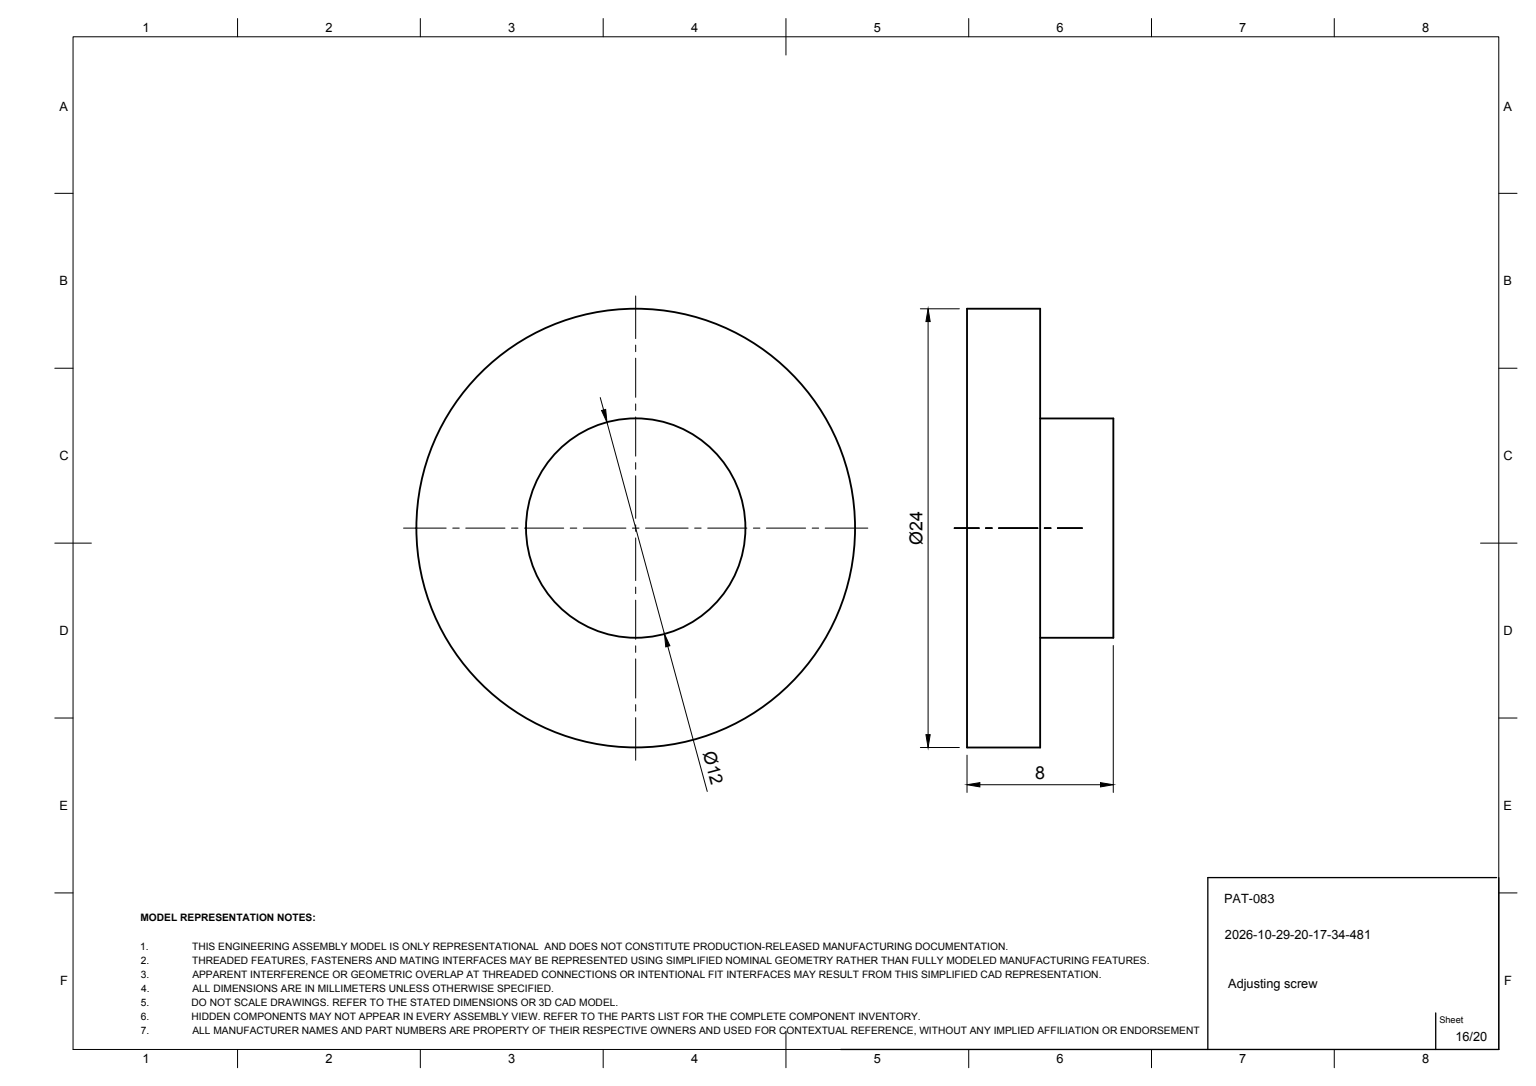
ISO-10303-21;
HEADER;
/* Generated by software containing ST-Developer
 * from STEP Tools, Inc. (www.steptools.com) 
 */

FILE_DESCRIPTION(
/* description */ ('PAT-083'),
/* implementation_level */ '2;1');

FILE_NAME(
/* name */ 'Adjusting screw.step',
/* time_stamp */ '2026-10-29T20:18:00-07:00',
/* author */ (''),
/* organization */ (''),
/* preprocessor_version */ 'ST-DEVELOPER v20.2',
/* originating_system */ 'Autodesk Translation Framework v15.17.0.0',
/* authorisation */ '');

FILE_SCHEMA (('AUTOMOTIVE_DESIGN { 1 0 10303 214 3 1 1 }'));
ENDSEC;

DATA;
#10=MECHANICAL_DESIGN_GEOMETRIC_PRESENTATION_REPRESENTATION('',(#243),#8428);
#195=SHAPE_REPRESENTATION_RELATIONSHIP('SRR','None',#8529,#219);
#219=ADVANCED_BREP_SHAPE_REPRESENTATION('',(#267),#8418);
#243=STYLED_ITEM('',(#8712),#267);
#267=MANIFOLD_SOLID_BREP('Body1',#3689);
#426=PLANE('',#4256);
#427=PLANE('',#4257);
#630=FACE_OUTER_BOUND('',#929,.T.);
#631=FACE_OUTER_BOUND('',#930,.T.);
#632=FACE_OUTER_BOUND('',#931,.T.);
#929=EDGE_LOOP('',(#2978,#2979,#2980,#2981));
#930=EDGE_LOOP('',(#2982));
#931=EDGE_LOOP('',(#2983));
#1153=LINE('',#7851,#1397);
#1397=VECTOR('',#5125,0.4);
#1668=CIRCLE('',#4254,0.4);
#1669=CIRCLE('',#4255,0.4);
#1881=VERTEX_POINT('',#7848);
#1882=VERTEX_POINT('',#7850);
#2265=EDGE_CURVE('',#1881,#1881,#1668,.T.);
#2266=EDGE_CURVE('',#1881,#1882,#1153,.T.);
#2267=EDGE_CURVE('',#1882,#1882,#1669,.T.);
#2978=ORIENTED_EDGE('',*,*,#2265,.F.);
#2979=ORIENTED_EDGE('',*,*,#2266,.T.);
#2980=ORIENTED_EDGE('',*,*,#2267,.T.);
#2981=ORIENTED_EDGE('',*,*,#2266,.F.);
#2982=ORIENTED_EDGE('',*,*,#2265,.T.);
#2983=ORIENTED_EDGE('',*,*,#2267,.F.);
#3427=CYLINDRICAL_SURFACE('',#4253,0.4);
#3577=ADVANCED_FACE('',(#630),#3427,.T.);
#3578=ADVANCED_FACE('',(#631),#426,.T.);
#3579=ADVANCED_FACE('',(#632),#427,.F.);
#3689=CLOSED_SHELL('',(#3577,#3578,#3579));
#4252=AXIS2_PLACEMENT_3D('',#7846,#5119,#5120);
#4253=AXIS2_PLACEMENT_3D('',#7847,#5121,#5122);
#4254=AXIS2_PLACEMENT_3D('',#7849,#5123,#5124);
#4255=AXIS2_PLACEMENT_3D('',#7852,#5126,#5127);
#4256=AXIS2_PLACEMENT_3D('',#7853,#5128,#5129);
#4257=AXIS2_PLACEMENT_3D('',#7854,#5130,#5131);
#5119=DIRECTION('axis',(0.,0.,1.));
#5120=DIRECTION('refdir',(1.,0.,0.));
#5121=DIRECTION('center_axis',(0.,0.,1.));
#5122=DIRECTION('ref_axis',(1.,0.,0.));
#5123=DIRECTION('center_axis',(0.,0.,1.));
#5124=DIRECTION('ref_axis',(1.,0.,0.));
#5125=DIRECTION('',(0.,0.,-1.));
#5126=DIRECTION('center_axis',(0.,0.,1.));
#5127=DIRECTION('ref_axis',(1.,0.,0.));
#5128=DIRECTION('center_axis',(0.,0.,1.));
#5129=DIRECTION('ref_axis',(1.,0.,0.));
#5130=DIRECTION('center_axis',(0.,0.,1.));
#5131=DIRECTION('ref_axis',(1.,0.,0.));
#7846=CARTESIAN_POINT('',(0.,0.,0.));
#7847=CARTESIAN_POINT('Origin',(0.,0.,8.));
#7848=CARTESIAN_POINT('',(-0.4,-4.89858719658941E-17,11.));
#7849=CARTESIAN_POINT('Origin',(0.,0.,11.));
#7850=CARTESIAN_POINT('',(-0.4,-4.89858719658941E-17,8.));
#7851=CARTESIAN_POINT('',(-0.4,-4.89858719658941E-17,8.));
#7852=CARTESIAN_POINT('Origin',(0.,0.,8.));
#7853=CARTESIAN_POINT('Origin',(0.,0.,11.));
#7854=CARTESIAN_POINT('Origin',(0.,0.,8.));
#8392=UNCERTAINTY_MEASURE_WITH_UNIT(LENGTH_MEASURE(0.001),#8429,
'DISTANCE_ACCURACY_VALUE',
'Maximum model space distance between geometric entities at asserted c
onnectivities');
#8402=UNCERTAINTY_MEASURE_WITH_UNIT(LENGTH_MEASURE(0.001),#8429,
'DISTANCE_ACCURACY_VALUE',
'Maximum model space distance between geometric entities at asserted c
onnectivities');
#8418=(
GEOMETRIC_REPRESENTATION_CONTEXT(3)
GLOBAL_UNCERTAINTY_ASSIGNED_CONTEXT((#8392))
GLOBAL_UNIT_ASSIGNED_CONTEXT((#8429,#8431,#8432))
REPRESENTATION_CONTEXT('','3D')
);
#8428=(
GEOMETRIC_REPRESENTATION_CONTEXT(3)
GLOBAL_UNCERTAINTY_ASSIGNED_CONTEXT((#8402))
GLOBAL_UNIT_ASSIGNED_CONTEXT((#8429,#8431,#8432))
REPRESENTATION_CONTEXT('','3D')
);
#8429=(
LENGTH_UNIT()
NAMED_UNIT(*)
SI_UNIT(.CENTI.,.METRE.)
);
#8431=(
NAMED_UNIT(*)
PLANE_ANGLE_UNIT()
SI_UNIT($,.RADIAN.)
);
#8432=(
NAMED_UNIT(*)
SI_UNIT($,.STERADIAN.)
SOLID_ANGLE_UNIT()
);
#8448=SHAPE_DEFINITION_REPRESENTATION(#8473,#8529);
#8473=PRODUCT_DEFINITION_SHAPE('',$,#8555);
#8529=SHAPE_REPRESENTATION('',(#4252),#8418);
#8539=PRODUCT_DEFINITION_CONTEXT('part definition',#8616,'design');
#8555=PRODUCT_DEFINITION('Adjusting screw','Adjusting screw',#8580,
#8539);
#8580=PRODUCT_DEFINITION_FORMATION('',$,#8633);
#8616=APPLICATION_CONTEXT(
'Core Data for Automotive Mechanical Design Process');
#8617=PRODUCT_CONTEXT('part definition',#8616,'mechanical');
#8633=PRODUCT('Adjusting screw','Adjusting screw',
'Adjusting screw',(#8617));
#8706=COLOUR_RGB('Black',0.12,0.14,0.17);
#8707=FILL_AREA_STYLE_COLOUR('',#8706);
#8708=FILL_AREA_STYLE('',(#8707));
#8709=SURFACE_STYLE_FILL_AREA(#8708);
#8710=SURFACE_SIDE_STYLE('',(#8709));
#8711=SURFACE_STYLE_USAGE(.BOTH.,#8710);
#8712=PRESENTATION_STYLE_ASSIGNMENT((#8711));
ENDSEC;
END-ISO-10303-21;
